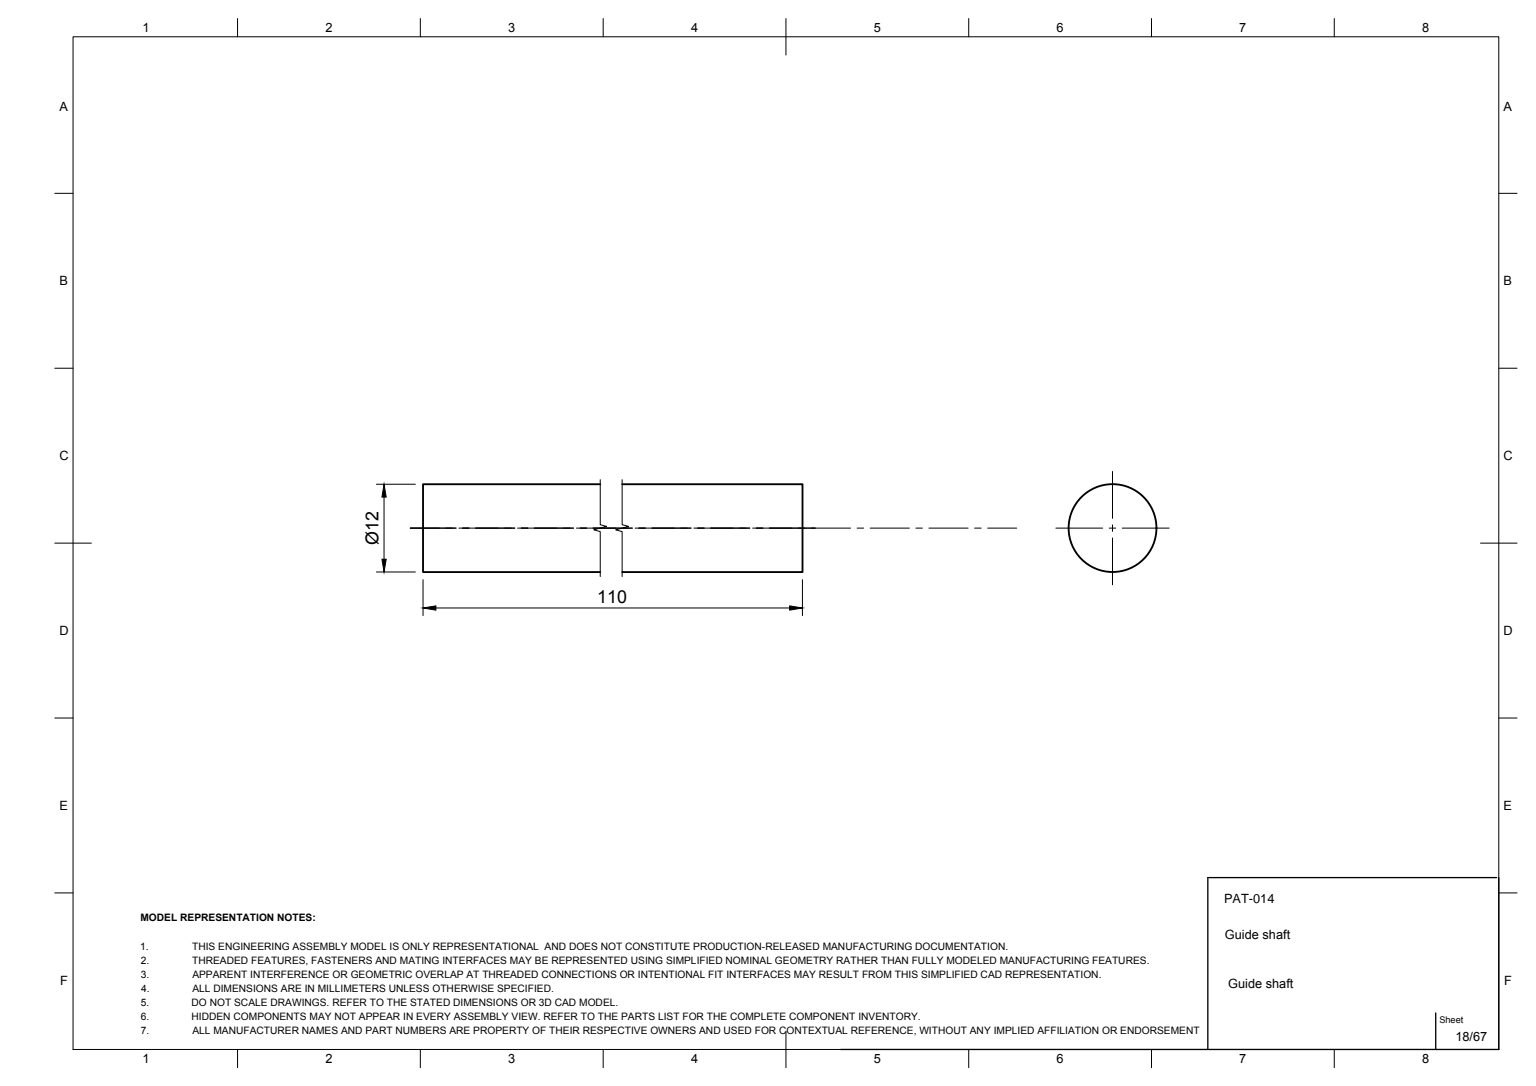
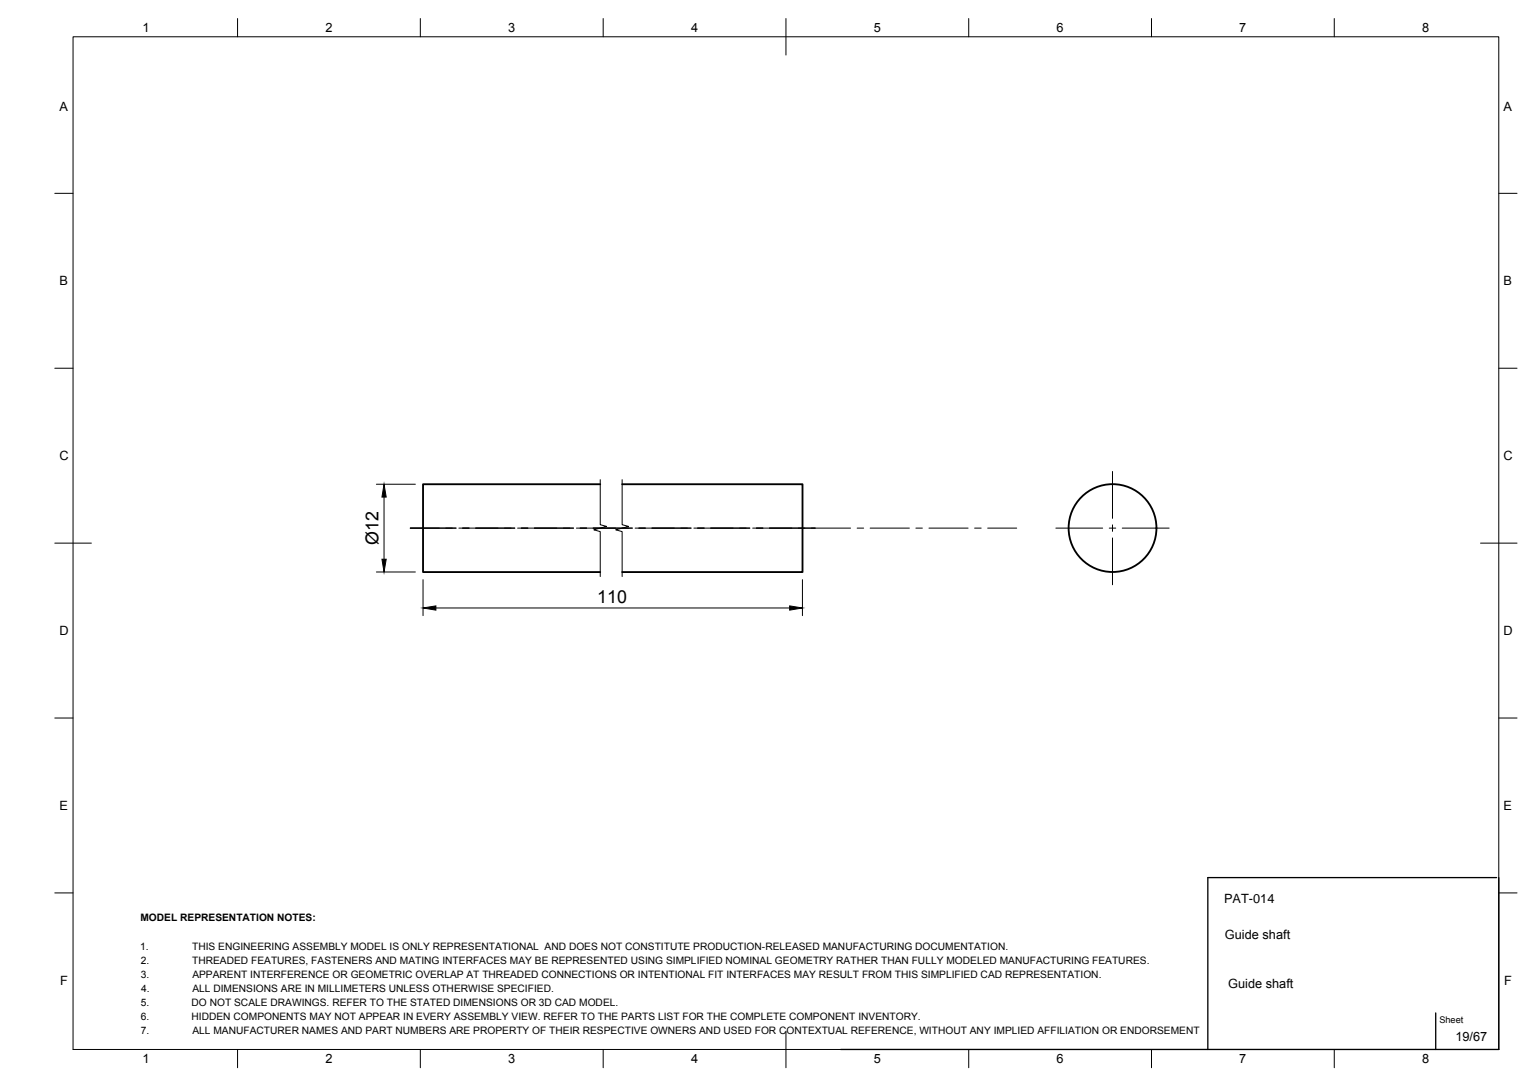
ISO-10303-21;
HEADER;
/* Generated by software containing ST-Developer
 * from STEP Tools, Inc. (www.steptools.com) 
 */

FILE_DESCRIPTION(
/* description */ ('Bin tilter linkage'),
/* implementation_level */ '2;1');

FILE_NAME(
/* name */ 'Guide shaft.step',
/* time_stamp */ '2026-10-28T03:26:24-07:00',
/* author */ (''),
/* organization */ (''),
/* preprocessor_version */ 'ST-DEVELOPER v20.2',
/* originating_system */ 'Autodesk Translation Framework v15.17.0.0',
/* authorisation */ '');

FILE_SCHEMA (('AUTOMOTIVE_DESIGN { 1 0 10303 214 3 1 1 }'));
ENDSEC;

DATA;
#10=MECHANICAL_DESIGN_GEOMETRIC_PRESENTATION_REPRESENTATION('',(#889),#23728);
#677=SHAPE_REPRESENTATION_RELATIONSHIP('SRR','None',#24141,#783);
#783=ADVANCED_BREP_SHAPE_REPRESENTATION('',(#1003),#23641);
#889=STYLED_ITEM('',(#24765),#1003);
#1003=MANIFOLD_SOLID_BREP('Body1',#12419);
#1602=PLANE('',#14167);
#1603=PLANE('',#14168);
#2116=FACE_OUTER_BOUND('',#3039,.T.);
#2117=FACE_OUTER_BOUND('',#3040,.T.);
#2118=FACE_OUTER_BOUND('',#3041,.T.);
#3039=EDGE_LOOP('',(#9297,#9298,#9299,#9300));
#3040=EDGE_LOOP('',(#9301));
#3041=EDGE_LOOP('',(#9302));
#4079=LINE('',#20775,#4754);
#4754=VECTOR('',#16684,0.6);
#5431=CIRCLE('',#14165,0.6);
#5432=CIRCLE('',#14166,0.6);
#6265=VERTEX_POINT('',#20772);
#6266=VERTEX_POINT('',#20774);
#7388=EDGE_CURVE('',#6265,#6265,#5431,.T.);
#7389=EDGE_CURVE('',#6265,#6266,#4079,.T.);
#7390=EDGE_CURVE('',#6266,#6266,#5432,.T.);
#9297=ORIENTED_EDGE('',*,*,#7388,.F.);
#9298=ORIENTED_EDGE('',*,*,#7389,.T.);
#9299=ORIENTED_EDGE('',*,*,#7390,.T.);
#9300=ORIENTED_EDGE('',*,*,#7389,.F.);
#9301=ORIENTED_EDGE('',*,*,#7388,.T.);
#9302=ORIENTED_EDGE('',*,*,#7390,.F.);
#11383=CYLINDRICAL_SURFACE('',#14164,0.6);
#11841=ADVANCED_FACE('',(#2116),#11383,.T.);
#11842=ADVANCED_FACE('',(#2117),#1602,.T.);
#11843=ADVANCED_FACE('',(#2118),#1603,.F.);
#12419=CLOSED_SHELL('',(#11841,#11842,#11843));
#14163=AXIS2_PLACEMENT_3D('',#20770,#16678,#16679);
#14164=AXIS2_PLACEMENT_3D('',#20771,#16680,#16681);
#14165=AXIS2_PLACEMENT_3D('',#20773,#16682,#16683);
#14166=AXIS2_PLACEMENT_3D('',#20776,#16685,#16686);
#14167=AXIS2_PLACEMENT_3D('',#20777,#16687,#16688);
#14168=AXIS2_PLACEMENT_3D('',#20778,#16689,#16690);
#16678=DIRECTION('axis',(0.,0.,1.));
#16679=DIRECTION('refdir',(1.,0.,0.));
#16680=DIRECTION('center_axis',(1.,0.,0.));
#16681=DIRECTION('ref_axis',(0.,0.,-1.));
#16682=DIRECTION('center_axis',(1.,0.,0.));
#16683=DIRECTION('ref_axis',(0.,0.,-1.));
#16684=DIRECTION('',(-1.,0.,0.));
#16685=DIRECTION('center_axis',(1.,0.,0.));
#16686=DIRECTION('ref_axis',(0.,0.,-1.));
#16687=DIRECTION('center_axis',(1.,0.,0.));
#16688=DIRECTION('ref_axis',(0.,0.,-1.));
#16689=DIRECTION('center_axis',(1.,0.,0.));
#16690=DIRECTION('ref_axis',(0.,0.,-1.));
#20770=CARTESIAN_POINT('',(0.,0.,0.));
#20771=CARTESIAN_POINT('Origin',(-10.,-7.,8.));
#20772=CARTESIAN_POINT('',(1.,-7.,8.6));
#20773=CARTESIAN_POINT('Origin',(1.,-7.,8.));
#20774=CARTESIAN_POINT('',(-10.,-7.,8.6));
#20775=CARTESIAN_POINT('',(-10.,-7.,8.6));
#20776=CARTESIAN_POINT('Origin',(-10.,-7.,8.));
#20777=CARTESIAN_POINT('Origin',(1.,-7.,8.));
#20778=CARTESIAN_POINT('Origin',(-10.,-7.,8.));
#23524=UNCERTAINTY_MEASURE_WITH_UNIT(LENGTH_MEASURE(0.001),#23729,
'DISTANCE_ACCURACY_VALUE',
'Maximum model space distance between geometric entities at asserted c
onnectivities');
#23611=UNCERTAINTY_MEASURE_WITH_UNIT(LENGTH_MEASURE(0.001),#23729,
'DISTANCE_ACCURACY_VALUE',
'Maximum model space distance between geometric entities at asserted c
onnectivities');
#23641=(
GEOMETRIC_REPRESENTATION_CONTEXT(3)
GLOBAL_UNCERTAINTY_ASSIGNED_CONTEXT((#23524))
GLOBAL_UNIT_ASSIGNED_CONTEXT((#23729,#23731,#23732))
REPRESENTATION_CONTEXT('','3D')
);
#23728=(
GEOMETRIC_REPRESENTATION_CONTEXT(3)
GLOBAL_UNCERTAINTY_ASSIGNED_CONTEXT((#23611))
GLOBAL_UNIT_ASSIGNED_CONTEXT((#23729,#23731,#23732))
REPRESENTATION_CONTEXT('','3D')
);
#23729=(
LENGTH_UNIT()
NAMED_UNIT(*)
SI_UNIT(.CENTI.,.METRE.)
);
#23731=(
NAMED_UNIT(*)
PLANE_ANGLE_UNIT()
SI_UNIT($,.RADIAN.)
);
#23732=(
NAMED_UNIT(*)
SI_UNIT($,.STERADIAN.)
SOLID_ANGLE_UNIT()
);
#23762=SHAPE_DEFINITION_REPRESENTATION(#23878,#24141);
#23878=PRODUCT_DEFINITION_SHAPE('',$,#24258);
#24141=SHAPE_REPRESENTATION('',(#14163),#23641);
#24228=PRODUCT_DEFINITION_CONTEXT('part definition',#24578,'design');
#24258=PRODUCT_DEFINITION('Guide shaft','Guide shaft',#24374,#24228);
#24374=PRODUCT_DEFINITION_FORMATION('',$,#24609);
#24578=APPLICATION_CONTEXT(
'Core Data for Automotive Mechanical Design Process');
#24579=PRODUCT_CONTEXT('part definition',#24578,'mechanical');
#24609=PRODUCT('Guide shaft','Guide shaft','Guide shaft',(#24579));
#24759=COLOUR_RGB('Grey',0.48,0.52,0.57);
#24760=FILL_AREA_STYLE_COLOUR('',#24759);
#24761=FILL_AREA_STYLE('',(#24760));
#24762=SURFACE_STYLE_FILL_AREA(#24761);
#24763=SURFACE_SIDE_STYLE('',(#24762));
#24764=SURFACE_STYLE_USAGE(.BOTH.,#24763);
#24765=PRESENTATION_STYLE_ASSIGNMENT((#24764));
ENDSEC;
END-ISO-10303-21;
